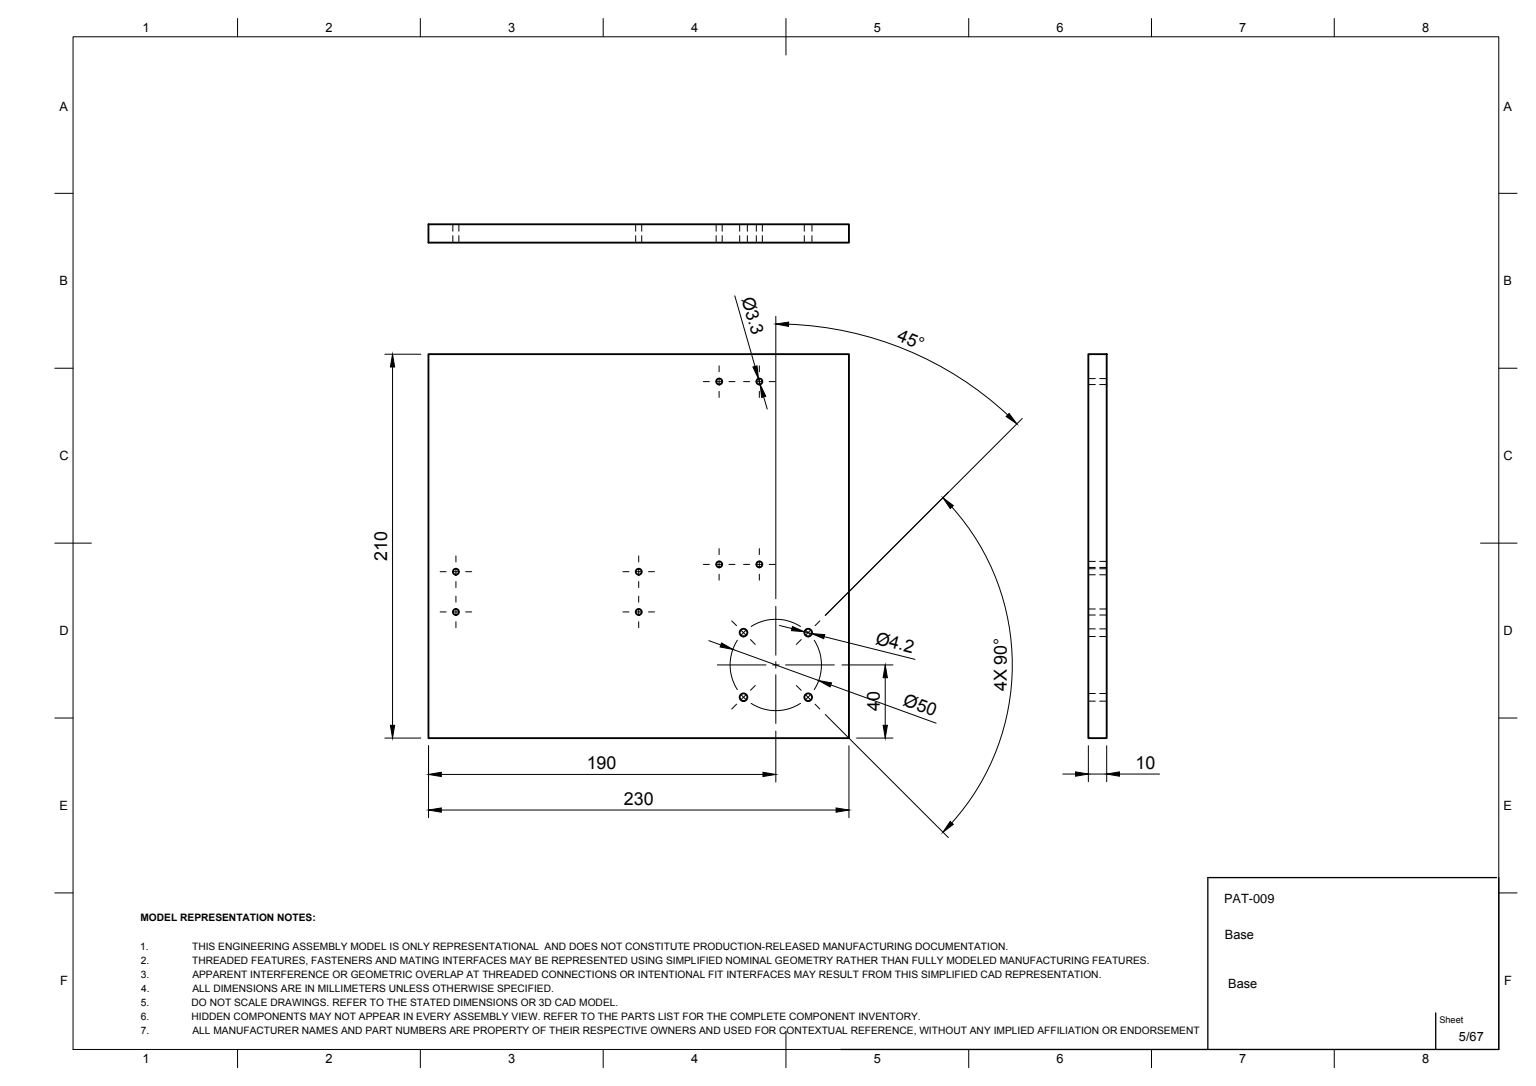
ISO-10303-21;
HEADER;
/* Generated by software containing ST-Developer
 * from STEP Tools, Inc. (www.steptools.com) 
 */

FILE_DESCRIPTION(
/* description */ ('Bell-crank linkage with push rods'),
/* implementation_level */ '2;1');

FILE_NAME(
/* name */ 'Base.step',
/* time_stamp */ '2026-10-28T03:25:15-07:00',
/* author */ (''),
/* organization */ (''),
/* preprocessor_version */ 'ST-DEVELOPER v20.2',
/* originating_system */ 'Autodesk Translation Framework v15.17.0.0',
/* authorisation */ '');

FILE_SCHEMA (('AUTOMOTIVE_DESIGN { 1 0 10303 214 3 1 1 }'));
ENDSEC;

DATA;
#10=MECHANICAL_DESIGN_GEOMETRIC_PRESENTATION_REPRESENTATION('',(#604),#16678);
#496=SHAPE_REPRESENTATION_RELATIONSHIP('SRR','None',#16912,#550);
#550=ADVANCED_BREP_SHAPE_REPRESENTATION('',(#666),#16617);
#604=STYLED_ITEM('',(#17270),#666);
#666=MANIFOLD_SOLID_BREP('Body1',#8794);
#725=FACE_BOUND('',#1786,.T.);
#726=FACE_BOUND('',#1787,.T.);
#727=FACE_BOUND('',#1788,.T.);
#728=FACE_BOUND('',#1789,.T.);
#729=FACE_BOUND('',#1790,.T.);
#730=FACE_BOUND('',#1791,.T.);
#731=FACE_BOUND('',#1792,.T.);
#732=FACE_BOUND('',#1793,.T.);
#733=FACE_BOUND('',#1794,.T.);
#734=FACE_BOUND('',#1795,.T.);
#735=FACE_BOUND('',#1796,.T.);
#736=FACE_BOUND('',#1797,.T.);
#737=FACE_BOUND('',#1799,.T.);
#738=FACE_BOUND('',#1800,.T.);
#739=FACE_BOUND('',#1801,.T.);
#740=FACE_BOUND('',#1802,.T.);
#741=FACE_BOUND('',#1803,.T.);
#742=FACE_BOUND('',#1804,.T.);
#743=FACE_BOUND('',#1805,.T.);
#744=FACE_BOUND('',#1806,.T.);
#745=FACE_BOUND('',#1807,.T.);
#746=FACE_BOUND('',#1808,.T.);
#747=FACE_BOUND('',#1809,.T.);
#748=FACE_BOUND('',#1810,.T.);
#966=PLANE('',#9493);
#967=PLANE('',#9494);
#968=PLANE('',#9495);
#969=PLANE('',#9496);
#970=PLANE('',#9497);
#971=PLANE('',#9498);
#1247=FACE_OUTER_BOUND('',#1769,.T.);
#1248=FACE_OUTER_BOUND('',#1770,.T.);
#1249=FACE_OUTER_BOUND('',#1771,.T.);
#1250=FACE_OUTER_BOUND('',#1772,.T.);
#1251=FACE_OUTER_BOUND('',#1773,.T.);
#1252=FACE_OUTER_BOUND('',#1774,.T.);
#1253=FACE_OUTER_BOUND('',#1775,.T.);
#1254=FACE_OUTER_BOUND('',#1776,.T.);
#1255=FACE_OUTER_BOUND('',#1777,.T.);
#1256=FACE_OUTER_BOUND('',#1778,.T.);
#1257=FACE_OUTER_BOUND('',#1779,.T.);
#1258=FACE_OUTER_BOUND('',#1780,.T.);
#1259=FACE_OUTER_BOUND('',#1781,.T.);
#1260=FACE_OUTER_BOUND('',#1782,.T.);
#1261=FACE_OUTER_BOUND('',#1783,.T.);
#1262=FACE_OUTER_BOUND('',#1784,.T.);
#1263=FACE_OUTER_BOUND('',#1785,.T.);
#1264=FACE_OUTER_BOUND('',#1798,.T.);
#1769=EDGE_LOOP('',(#5911,#5912,#5913,#5914));
#1770=EDGE_LOOP('',(#5915,#5916,#5917,#5918));
#1771=EDGE_LOOP('',(#5919,#5920,#5921,#5922));
#1772=EDGE_LOOP('',(#5923,#5924,#5925,#5926));
#1773=EDGE_LOOP('',(#5927,#5928,#5929,#5930));
#1774=EDGE_LOOP('',(#5931,#5932,#5933,#5934));
#1775=EDGE_LOOP('',(#5935,#5936,#5937,#5938));
#1776=EDGE_LOOP('',(#5939,#5940,#5941,#5942));
#1777=EDGE_LOOP('',(#5943,#5944,#5945,#5946));
#1778=EDGE_LOOP('',(#5947,#5948,#5949,#5950));
#1779=EDGE_LOOP('',(#5951,#5952,#5953,#5954));
#1780=EDGE_LOOP('',(#5955,#5956,#5957,#5958));
#1781=EDGE_LOOP('',(#5959,#5960,#5961,#5962));
#1782=EDGE_LOOP('',(#5963,#5964,#5965,#5966));
#1783=EDGE_LOOP('',(#5967,#5968,#5969,#5970));
#1784=EDGE_LOOP('',(#5971,#5972,#5973,#5974));
#1785=EDGE_LOOP('',(#5975,#5976,#5977,#5978));
#1786=EDGE_LOOP('',(#5979));
#1787=EDGE_LOOP('',(#5980));
#1788=EDGE_LOOP('',(#5981));
#1789=EDGE_LOOP('',(#5982));
#1790=EDGE_LOOP('',(#5983));
#1791=EDGE_LOOP('',(#5984));
#1792=EDGE_LOOP('',(#5985));
#1793=EDGE_LOOP('',(#5986));
#1794=EDGE_LOOP('',(#5987));
#1795=EDGE_LOOP('',(#5988));
#1796=EDGE_LOOP('',(#5989));
#1797=EDGE_LOOP('',(#5990));
#1798=EDGE_LOOP('',(#5991,#5992,#5993,#5994));
#1799=EDGE_LOOP('',(#5995));
#1800=EDGE_LOOP('',(#5996));
#1801=EDGE_LOOP('',(#5997));
#1802=EDGE_LOOP('',(#5998));
#1803=EDGE_LOOP('',(#5999));
#1804=EDGE_LOOP('',(#6000));
#1805=EDGE_LOOP('',(#6001));
#1806=EDGE_LOOP('',(#6002));
#1807=EDGE_LOOP('',(#6003));
#1808=EDGE_LOOP('',(#6004));
#1809=EDGE_LOOP('',(#6005));
#1810=EDGE_LOOP('',(#6006));
#2532=LINE('',#13538,#3081);
#2533=LINE('',#13544,#3082);
#2534=LINE('',#13550,#3083);
#2535=LINE('',#13556,#3084);
#2536=LINE('',#13562,#3085);
#2537=LINE('',#13568,#3086);
#2538=LINE('',#13574,#3087);
#2539=LINE('',#13580,#3088);
#2540=LINE('',#13586,#3089);
#2541=LINE('',#13592,#3090);
#2542=LINE('',#13598,#3091);
#2543=LINE('',#13604,#3092);
#2544=LINE('',#13609,#3093);
#2545=LINE('',#13611,#3094);
#2546=LINE('',#13613,#3095);
#2547=LINE('',#13614,#3096);
#2548=LINE('',#13617,#3097);
#2549=LINE('',#13619,#3098);
#2550=LINE('',#13620,#3099);
#2551=LINE('',#13623,#3100);
#2552=LINE('',#13625,#3101);
#2553=LINE('',#13626,#3102);
#2554=LINE('',#13628,#3103);
#2555=LINE('',#13629,#3104);
#3081=VECTOR('',#10640,0.165);
#3082=VECTOR('',#10647,0.165);
#3083=VECTOR('',#10654,0.165);
#3084=VECTOR('',#10661,0.165);
#3085=VECTOR('',#10668,0.164999999999999);
#3086=VECTOR('',#10675,0.164999999999999);
#3087=VECTOR('',#10682,0.165);
#3088=VECTOR('',#10689,0.165);
#3089=VECTOR('',#10696,0.21);
#3090=VECTOR('',#10703,0.21);
#3091=VECTOR('',#10710,0.21);
#3092=VECTOR('',#10717,0.21);
#3093=VECTOR('',#10722,1.);
#3094=VECTOR('',#10723,1.);
#3095=VECTOR('',#10724,1.);
#3096=VECTOR('',#10725,1.);
#3097=VECTOR('',#10728,1.);
#3098=VECTOR('',#10729,1.);
#3099=VECTOR('',#10730,1.);
#3100=VECTOR('',#10733,1.);
#3101=VECTOR('',#10734,1.);
#3102=VECTOR('',#10735,1.);
#3103=VECTOR('',#10738,1.);
#3104=VECTOR('',#10739,1.);
#3630=CIRCLE('',#9458,0.165);
#3631=CIRCLE('',#9459,0.165);
#3632=CIRCLE('',#9461,0.165);
#3633=CIRCLE('',#9462,0.165);
#3634=CIRCLE('',#9464,0.165);
#3635=CIRCLE('',#9465,0.165);
#3636=CIRCLE('',#9467,0.165);
#3637=CIRCLE('',#9468,0.165);
#3638=CIRCLE('',#9470,0.164999999999999);
#3639=CIRCLE('',#9471,0.164999999999999);
#3640=CIRCLE('',#9473,0.164999999999999);
#3641=CIRCLE('',#9474,0.164999999999999);
#3642=CIRCLE('',#9476,0.165);
#3643=CIRCLE('',#9477,0.165);
#3644=CIRCLE('',#9479,0.165);
#3645=CIRCLE('',#9480,0.165);
#3646=CIRCLE('',#9482,0.21);
#3647=CIRCLE('',#9483,0.21);
#3648=CIRCLE('',#9485,0.21);
#3649=CIRCLE('',#9486,0.21);
#3650=CIRCLE('',#9488,0.21);
#3651=CIRCLE('',#9489,0.21);
#3652=CIRCLE('',#9491,0.21);
#3653=CIRCLE('',#9492,0.21);
#4120=VERTEX_POINT('',#13535);
#4121=VERTEX_POINT('',#13537);
#4122=VERTEX_POINT('',#13541);
#4123=VERTEX_POINT('',#13543);
#4124=VERTEX_POINT('',#13547);
#4125=VERTEX_POINT('',#13549);
#4126=VERTEX_POINT('',#13553);
#4127=VERTEX_POINT('',#13555);
#4128=VERTEX_POINT('',#13559);
#4129=VERTEX_POINT('',#13561);
#4130=VERTEX_POINT('',#13565);
#4131=VERTEX_POINT('',#13567);
#4132=VERTEX_POINT('',#13571);
#4133=VERTEX_POINT('',#13573);
#4134=VERTEX_POINT('',#13577);
#4135=VERTEX_POINT('',#13579);
#4136=VERTEX_POINT('',#13583);
#4137=VERTEX_POINT('',#13585);
#4138=VERTEX_POINT('',#13589);
#4139=VERTEX_POINT('',#13591);
#4140=VERTEX_POINT('',#13595);
#4141=VERTEX_POINT('',#13597);
#4142=VERTEX_POINT('',#13601);
#4143=VERTEX_POINT('',#13603);
#4144=VERTEX_POINT('',#13607);
#4145=VERTEX_POINT('',#13608);
#4146=VERTEX_POINT('',#13610);
#4147=VERTEX_POINT('',#13612);
#4148=VERTEX_POINT('',#13616);
#4149=VERTEX_POINT('',#13618);
#4150=VERTEX_POINT('',#13622);
#4151=VERTEX_POINT('',#13624);
#4833=EDGE_CURVE('',#4120,#4120,#3630,.T.);
#4834=EDGE_CURVE('',#4120,#4121,#2532,.T.);
#4835=EDGE_CURVE('',#4121,#4121,#3631,.T.);
#4836=EDGE_CURVE('',#4122,#4122,#3632,.T.);
#4837=EDGE_CURVE('',#4122,#4123,#2533,.T.);
#4838=EDGE_CURVE('',#4123,#4123,#3633,.T.);
#4839=EDGE_CURVE('',#4124,#4124,#3634,.T.);
#4840=EDGE_CURVE('',#4124,#4125,#2534,.T.);
#4841=EDGE_CURVE('',#4125,#4125,#3635,.T.);
#4842=EDGE_CURVE('',#4126,#4126,#3636,.T.);
#4843=EDGE_CURVE('',#4126,#4127,#2535,.T.);
#4844=EDGE_CURVE('',#4127,#4127,#3637,.T.);
#4845=EDGE_CURVE('',#4128,#4128,#3638,.T.);
#4846=EDGE_CURVE('',#4128,#4129,#2536,.T.);
#4847=EDGE_CURVE('',#4129,#4129,#3639,.T.);
#4848=EDGE_CURVE('',#4130,#4130,#3640,.T.);
#4849=EDGE_CURVE('',#4130,#4131,#2537,.T.);
#4850=EDGE_CURVE('',#4131,#4131,#3641,.T.);
#4851=EDGE_CURVE('',#4132,#4132,#3642,.T.);
#4852=EDGE_CURVE('',#4132,#4133,#2538,.T.);
#4853=EDGE_CURVE('',#4133,#4133,#3643,.T.);
#4854=EDGE_CURVE('',#4134,#4134,#3644,.T.);
#4855=EDGE_CURVE('',#4134,#4135,#2539,.T.);
#4856=EDGE_CURVE('',#4135,#4135,#3645,.T.);
#4857=EDGE_CURVE('',#4136,#4136,#3646,.T.);
#4858=EDGE_CURVE('',#4136,#4137,#2540,.T.);
#4859=EDGE_CURVE('',#4137,#4137,#3647,.T.);
#4860=EDGE_CURVE('',#4138,#4138,#3648,.T.);
#4861=EDGE_CURVE('',#4138,#4139,#2541,.T.);
#4862=EDGE_CURVE('',#4139,#4139,#3649,.T.);
#4863=EDGE_CURVE('',#4140,#4140,#3650,.T.);
#4864=EDGE_CURVE('',#4140,#4141,#2542,.T.);
#4865=EDGE_CURVE('',#4141,#4141,#3651,.T.);
#4866=EDGE_CURVE('',#4142,#4142,#3652,.T.);
#4867=EDGE_CURVE('',#4142,#4143,#2543,.T.);
#4868=EDGE_CURVE('',#4143,#4143,#3653,.T.);
#4869=EDGE_CURVE('',#4144,#4145,#2544,.T.);
#4870=EDGE_CURVE('',#4145,#4146,#2545,.T.);
#4871=EDGE_CURVE('',#4147,#4146,#2546,.T.);
#4872=EDGE_CURVE('',#4144,#4147,#2547,.T.);
#4873=EDGE_CURVE('',#4148,#4144,#2548,.T.);
#4874=EDGE_CURVE('',#4149,#4147,#2549,.T.);
#4875=EDGE_CURVE('',#4148,#4149,#2550,.T.);
#4876=EDGE_CURVE('',#4150,#4148,#2551,.T.);
#4877=EDGE_CURVE('',#4151,#4149,#2552,.T.);
#4878=EDGE_CURVE('',#4150,#4151,#2553,.T.);
#4879=EDGE_CURVE('',#4145,#4150,#2554,.T.);
#4880=EDGE_CURVE('',#4146,#4151,#2555,.T.);
#5911=ORIENTED_EDGE('',*,*,#4833,.F.);
#5912=ORIENTED_EDGE('',*,*,#4834,.T.);
#5913=ORIENTED_EDGE('',*,*,#4835,.F.);
#5914=ORIENTED_EDGE('',*,*,#4834,.F.);
#5915=ORIENTED_EDGE('',*,*,#4836,.F.);
#5916=ORIENTED_EDGE('',*,*,#4837,.T.);
#5917=ORIENTED_EDGE('',*,*,#4838,.F.);
#5918=ORIENTED_EDGE('',*,*,#4837,.F.);
#5919=ORIENTED_EDGE('',*,*,#4839,.F.);
#5920=ORIENTED_EDGE('',*,*,#4840,.T.);
#5921=ORIENTED_EDGE('',*,*,#4841,.F.);
#5922=ORIENTED_EDGE('',*,*,#4840,.F.);
#5923=ORIENTED_EDGE('',*,*,#4842,.F.);
#5924=ORIENTED_EDGE('',*,*,#4843,.T.);
#5925=ORIENTED_EDGE('',*,*,#4844,.F.);
#5926=ORIENTED_EDGE('',*,*,#4843,.F.);
#5927=ORIENTED_EDGE('',*,*,#4845,.F.);
#5928=ORIENTED_EDGE('',*,*,#4846,.T.);
#5929=ORIENTED_EDGE('',*,*,#4847,.F.);
#5930=ORIENTED_EDGE('',*,*,#4846,.F.);
#5931=ORIENTED_EDGE('',*,*,#4848,.F.);
#5932=ORIENTED_EDGE('',*,*,#4849,.T.);
#5933=ORIENTED_EDGE('',*,*,#4850,.F.);
#5934=ORIENTED_EDGE('',*,*,#4849,.F.);
#5935=ORIENTED_EDGE('',*,*,#4851,.F.);
#5936=ORIENTED_EDGE('',*,*,#4852,.T.);
#5937=ORIENTED_EDGE('',*,*,#4853,.F.);
#5938=ORIENTED_EDGE('',*,*,#4852,.F.);
#5939=ORIENTED_EDGE('',*,*,#4854,.F.);
#5940=ORIENTED_EDGE('',*,*,#4855,.T.);
#5941=ORIENTED_EDGE('',*,*,#4856,.F.);
#5942=ORIENTED_EDGE('',*,*,#4855,.F.);
#5943=ORIENTED_EDGE('',*,*,#4857,.F.);
#5944=ORIENTED_EDGE('',*,*,#4858,.T.);
#5945=ORIENTED_EDGE('',*,*,#4859,.F.);
#5946=ORIENTED_EDGE('',*,*,#4858,.F.);
#5947=ORIENTED_EDGE('',*,*,#4860,.F.);
#5948=ORIENTED_EDGE('',*,*,#4861,.T.);
#5949=ORIENTED_EDGE('',*,*,#4862,.F.);
#5950=ORIENTED_EDGE('',*,*,#4861,.F.);
#5951=ORIENTED_EDGE('',*,*,#4863,.F.);
#5952=ORIENTED_EDGE('',*,*,#4864,.T.);
#5953=ORIENTED_EDGE('',*,*,#4865,.F.);
#5954=ORIENTED_EDGE('',*,*,#4864,.F.);
#5955=ORIENTED_EDGE('',*,*,#4866,.F.);
#5956=ORIENTED_EDGE('',*,*,#4867,.T.);
#5957=ORIENTED_EDGE('',*,*,#4868,.F.);
#5958=ORIENTED_EDGE('',*,*,#4867,.F.);
#5959=ORIENTED_EDGE('',*,*,#4869,.T.);
#5960=ORIENTED_EDGE('',*,*,#4870,.T.);
#5961=ORIENTED_EDGE('',*,*,#4871,.F.);
#5962=ORIENTED_EDGE('',*,*,#4872,.F.);
#5963=ORIENTED_EDGE('',*,*,#4873,.T.);
#5964=ORIENTED_EDGE('',*,*,#4872,.T.);
#5965=ORIENTED_EDGE('',*,*,#4874,.F.);
#5966=ORIENTED_EDGE('',*,*,#4875,.F.);
#5967=ORIENTED_EDGE('',*,*,#4876,.T.);
#5968=ORIENTED_EDGE('',*,*,#4875,.T.);
#5969=ORIENTED_EDGE('',*,*,#4877,.F.);
#5970=ORIENTED_EDGE('',*,*,#4878,.F.);
#5971=ORIENTED_EDGE('',*,*,#4879,.T.);
#5972=ORIENTED_EDGE('',*,*,#4878,.T.);
#5973=ORIENTED_EDGE('',*,*,#4880,.F.);
#5974=ORIENTED_EDGE('',*,*,#4870,.F.);
#5975=ORIENTED_EDGE('',*,*,#4880,.T.);
#5976=ORIENTED_EDGE('',*,*,#4877,.T.);
#5977=ORIENTED_EDGE('',*,*,#4874,.T.);
#5978=ORIENTED_EDGE('',*,*,#4871,.T.);
#5979=ORIENTED_EDGE('',*,*,#4841,.T.);
#5980=ORIENTED_EDGE('',*,*,#4844,.T.);
#5981=ORIENTED_EDGE('',*,*,#4868,.T.);
#5982=ORIENTED_EDGE('',*,*,#4865,.T.);
#5983=ORIENTED_EDGE('',*,*,#4862,.T.);
#5984=ORIENTED_EDGE('',*,*,#4859,.T.);
#5985=ORIENTED_EDGE('',*,*,#4856,.T.);
#5986=ORIENTED_EDGE('',*,*,#4853,.T.);
#5987=ORIENTED_EDGE('',*,*,#4850,.T.);
#5988=ORIENTED_EDGE('',*,*,#4847,.T.);
#5989=ORIENTED_EDGE('',*,*,#4838,.T.);
#5990=ORIENTED_EDGE('',*,*,#4835,.T.);
#5991=ORIENTED_EDGE('',*,*,#4879,.F.);
#5992=ORIENTED_EDGE('',*,*,#4869,.F.);
#5993=ORIENTED_EDGE('',*,*,#4873,.F.);
#5994=ORIENTED_EDGE('',*,*,#4876,.F.);
#5995=ORIENTED_EDGE('',*,*,#4839,.T.);
#5996=ORIENTED_EDGE('',*,*,#4842,.T.);
#5997=ORIENTED_EDGE('',*,*,#4866,.T.);
#5998=ORIENTED_EDGE('',*,*,#4863,.T.);
#5999=ORIENTED_EDGE('',*,*,#4860,.T.);
#6000=ORIENTED_EDGE('',*,*,#4857,.T.);
#6001=ORIENTED_EDGE('',*,*,#4854,.T.);
#6002=ORIENTED_EDGE('',*,*,#4851,.T.);
#6003=ORIENTED_EDGE('',*,*,#4848,.T.);
#6004=ORIENTED_EDGE('',*,*,#4845,.T.);
#6005=ORIENTED_EDGE('',*,*,#4836,.T.);
#6006=ORIENTED_EDGE('',*,*,#4833,.T.);
#8067=CYLINDRICAL_SURFACE('',#9457,0.165);
#8068=CYLINDRICAL_SURFACE('',#9460,0.165);
#8069=CYLINDRICAL_SURFACE('',#9463,0.165);
#8070=CYLINDRICAL_SURFACE('',#9466,0.165);
#8071=CYLINDRICAL_SURFACE('',#9469,0.164999999999999);
#8072=CYLINDRICAL_SURFACE('',#9472,0.164999999999999);
#8073=CYLINDRICAL_SURFACE('',#9475,0.165);
#8074=CYLINDRICAL_SURFACE('',#9478,0.165);
#8075=CYLINDRICAL_SURFACE('',#9481,0.21);
#8076=CYLINDRICAL_SURFACE('',#9484,0.21);
#8077=CYLINDRICAL_SURFACE('',#9487,0.21);
#8078=CYLINDRICAL_SURFACE('',#9490,0.21);
#8272=ADVANCED_FACE('',(#1247),#8067,.F.);
#8273=ADVANCED_FACE('',(#1248),#8068,.F.);
#8274=ADVANCED_FACE('',(#1249),#8069,.F.);
#8275=ADVANCED_FACE('',(#1250),#8070,.F.);
#8276=ADVANCED_FACE('',(#1251),#8071,.F.);
#8277=ADVANCED_FACE('',(#1252),#8072,.F.);
#8278=ADVANCED_FACE('',(#1253),#8073,.F.);
#8279=ADVANCED_FACE('',(#1254),#8074,.F.);
#8280=ADVANCED_FACE('',(#1255),#8075,.F.);
#8281=ADVANCED_FACE('',(#1256),#8076,.F.);
#8282=ADVANCED_FACE('',(#1257),#8077,.F.);
#8283=ADVANCED_FACE('',(#1258),#8078,.F.);
#8284=ADVANCED_FACE('',(#1259),#966,.T.);
#8285=ADVANCED_FACE('',(#1260),#967,.T.);
#8286=ADVANCED_FACE('',(#1261),#968,.T.);
#8287=ADVANCED_FACE('',(#1262),#969,.T.);
#8288=ADVANCED_FACE('',(#1263,#725,#726,#727,#728,#729,#730,#731,#732,#733,
#734,#735,#736),#970,.T.);
#8289=ADVANCED_FACE('',(#1264,#737,#738,#739,#740,#741,#742,#743,#744,#745,
#746,#747,#748),#971,.F.);
#8794=CLOSED_SHELL('',(#8272,#8273,#8274,#8275,#8276,#8277,#8278,#8279,
#8280,#8281,#8282,#8283,#8284,#8285,#8286,#8287,#8288,#8289));
#9456=AXIS2_PLACEMENT_3D('',#13533,#10634,#10635);
#9457=AXIS2_PLACEMENT_3D('',#13534,#10636,#10637);
#9458=AXIS2_PLACEMENT_3D('',#13536,#10638,#10639);
#9459=AXIS2_PLACEMENT_3D('',#13539,#10641,#10642);
#9460=AXIS2_PLACEMENT_3D('',#13540,#10643,#10644);
#9461=AXIS2_PLACEMENT_3D('',#13542,#10645,#10646);
#9462=AXIS2_PLACEMENT_3D('',#13545,#10648,#10649);
#9463=AXIS2_PLACEMENT_3D('',#13546,#10650,#10651);
#9464=AXIS2_PLACEMENT_3D('',#13548,#10652,#10653);
#9465=AXIS2_PLACEMENT_3D('',#13551,#10655,#10656);
#9466=AXIS2_PLACEMENT_3D('',#13552,#10657,#10658);
#9467=AXIS2_PLACEMENT_3D('',#13554,#10659,#10660);
#9468=AXIS2_PLACEMENT_3D('',#13557,#10662,#10663);
#9469=AXIS2_PLACEMENT_3D('',#13558,#10664,#10665);
#9470=AXIS2_PLACEMENT_3D('',#13560,#10666,#10667);
#9471=AXIS2_PLACEMENT_3D('',#13563,#10669,#10670);
#9472=AXIS2_PLACEMENT_3D('',#13564,#10671,#10672);
#9473=AXIS2_PLACEMENT_3D('',#13566,#10673,#10674);
#9474=AXIS2_PLACEMENT_3D('',#13569,#10676,#10677);
#9475=AXIS2_PLACEMENT_3D('',#13570,#10678,#10679);
#9476=AXIS2_PLACEMENT_3D('',#13572,#10680,#10681);
#9477=AXIS2_PLACEMENT_3D('',#13575,#10683,#10684);
#9478=AXIS2_PLACEMENT_3D('',#13576,#10685,#10686);
#9479=AXIS2_PLACEMENT_3D('',#13578,#10687,#10688);
#9480=AXIS2_PLACEMENT_3D('',#13581,#10690,#10691);
#9481=AXIS2_PLACEMENT_3D('',#13582,#10692,#10693);
#9482=AXIS2_PLACEMENT_3D('',#13584,#10694,#10695);
#9483=AXIS2_PLACEMENT_3D('',#13587,#10697,#10698);
#9484=AXIS2_PLACEMENT_3D('',#13588,#10699,#10700);
#9485=AXIS2_PLACEMENT_3D('',#13590,#10701,#10702);
#9486=AXIS2_PLACEMENT_3D('',#13593,#10704,#10705);
#9487=AXIS2_PLACEMENT_3D('',#13594,#10706,#10707);
#9488=AXIS2_PLACEMENT_3D('',#13596,#10708,#10709);
#9489=AXIS2_PLACEMENT_3D('',#13599,#10711,#10712);
#9490=AXIS2_PLACEMENT_3D('',#13600,#10713,#10714);
#9491=AXIS2_PLACEMENT_3D('',#13602,#10715,#10716);
#9492=AXIS2_PLACEMENT_3D('',#13605,#10718,#10719);
#9493=AXIS2_PLACEMENT_3D('',#13606,#10720,#10721);
#9494=AXIS2_PLACEMENT_3D('',#13615,#10726,#10727);
#9495=AXIS2_PLACEMENT_3D('',#13621,#10731,#10732);
#9496=AXIS2_PLACEMENT_3D('',#13627,#10736,#10737);
#9497=AXIS2_PLACEMENT_3D('',#13630,#10740,#10741);
#9498=AXIS2_PLACEMENT_3D('',#13631,#10742,#10743);
#10634=DIRECTION('axis',(0.,0.,1.));
#10635=DIRECTION('refdir',(1.,0.,0.));
#10636=DIRECTION('center_axis',(0.,0.,1.));
#10637=DIRECTION('ref_axis',(1.,0.,0.));
#10638=DIRECTION('center_axis',(0.,0.,1.));
#10639=DIRECTION('ref_axis',(1.,0.,0.));
#10640=DIRECTION('',(0.,0.,1.));
#10641=DIRECTION('center_axis',(0.,0.,-1.));
#10642=DIRECTION('ref_axis',(1.,0.,0.));
#10643=DIRECTION('center_axis',(0.,0.,1.));
#10644=DIRECTION('ref_axis',(1.,0.,0.));
#10645=DIRECTION('center_axis',(0.,0.,1.));
#10646=DIRECTION('ref_axis',(1.,0.,0.));
#10647=DIRECTION('',(0.,0.,1.));
#10648=DIRECTION('center_axis',(0.,0.,-1.));
#10649=DIRECTION('ref_axis',(1.,0.,0.));
#10650=DIRECTION('center_axis',(0.,0.,1.));
#10651=DIRECTION('ref_axis',(1.,0.,0.));
#10652=DIRECTION('center_axis',(0.,0.,1.));
#10653=DIRECTION('ref_axis',(1.,0.,0.));
#10654=DIRECTION('',(0.,0.,1.));
#10655=DIRECTION('center_axis',(0.,0.,-1.));
#10656=DIRECTION('ref_axis',(1.,0.,0.));
#10657=DIRECTION('center_axis',(0.,0.,1.));
#10658=DIRECTION('ref_axis',(1.,0.,0.));
#10659=DIRECTION('center_axis',(0.,0.,1.));
#10660=DIRECTION('ref_axis',(1.,0.,0.));
#10661=DIRECTION('',(0.,0.,1.));
#10662=DIRECTION('center_axis',(0.,0.,-1.));
#10663=DIRECTION('ref_axis',(1.,0.,0.));
#10664=DIRECTION('center_axis',(0.,0.,1.));
#10665=DIRECTION('ref_axis',(1.,0.,0.));
#10666=DIRECTION('center_axis',(0.,0.,1.));
#10667=DIRECTION('ref_axis',(1.,0.,0.));
#10668=DIRECTION('',(0.,0.,1.));
#10669=DIRECTION('center_axis',(0.,0.,-1.));
#10670=DIRECTION('ref_axis',(1.,0.,0.));
#10671=DIRECTION('center_axis',(0.,0.,1.));
#10672=DIRECTION('ref_axis',(1.,0.,0.));
#10673=DIRECTION('center_axis',(0.,0.,1.));
#10674=DIRECTION('ref_axis',(1.,0.,0.));
#10675=DIRECTION('',(0.,0.,1.));
#10676=DIRECTION('center_axis',(0.,0.,-1.));
#10677=DIRECTION('ref_axis',(1.,0.,0.));
#10678=DIRECTION('center_axis',(0.,0.,1.));
#10679=DIRECTION('ref_axis',(1.,0.,0.));
#10680=DIRECTION('center_axis',(0.,0.,1.));
#10681=DIRECTION('ref_axis',(1.,0.,0.));
#10682=DIRECTION('',(0.,0.,1.));
#10683=DIRECTION('center_axis',(0.,0.,-1.));
#10684=DIRECTION('ref_axis',(1.,0.,0.));
#10685=DIRECTION('center_axis',(0.,0.,1.));
#10686=DIRECTION('ref_axis',(1.,0.,0.));
#10687=DIRECTION('center_axis',(0.,0.,1.));
#10688=DIRECTION('ref_axis',(1.,0.,0.));
#10689=DIRECTION('',(0.,0.,1.));
#10690=DIRECTION('center_axis',(0.,0.,-1.));
#10691=DIRECTION('ref_axis',(1.,0.,0.));
#10692=DIRECTION('center_axis',(0.,0.,1.));
#10693=DIRECTION('ref_axis',(1.,0.,0.));
#10694=DIRECTION('center_axis',(0.,0.,1.));
#10695=DIRECTION('ref_axis',(1.,0.,0.));
#10696=DIRECTION('',(0.,0.,1.));
#10697=DIRECTION('center_axis',(0.,0.,-1.));
#10698=DIRECTION('ref_axis',(1.,0.,0.));
#10699=DIRECTION('center_axis',(0.,0.,1.));
#10700=DIRECTION('ref_axis',(1.,0.,0.));
#10701=DIRECTION('center_axis',(0.,0.,1.));
#10702=DIRECTION('ref_axis',(1.,0.,0.));
#10703=DIRECTION('',(0.,0.,1.));
#10704=DIRECTION('center_axis',(0.,0.,-1.));
#10705=DIRECTION('ref_axis',(1.,0.,0.));
#10706=DIRECTION('center_axis',(0.,0.,1.));
#10707=DIRECTION('ref_axis',(1.,0.,0.));
#10708=DIRECTION('center_axis',(0.,0.,1.));
#10709=DIRECTION('ref_axis',(1.,0.,0.));
#10710=DIRECTION('',(0.,0.,1.));
#10711=DIRECTION('center_axis',(0.,0.,-1.));
#10712=DIRECTION('ref_axis',(1.,0.,0.));
#10713=DIRECTION('center_axis',(0.,0.,1.));
#10714=DIRECTION('ref_axis',(1.,0.,0.));
#10715=DIRECTION('center_axis',(0.,0.,1.));
#10716=DIRECTION('ref_axis',(1.,0.,0.));
#10717=DIRECTION('',(0.,0.,1.));
#10718=DIRECTION('center_axis',(0.,0.,-1.));
#10719=DIRECTION('ref_axis',(1.,0.,0.));
#10720=DIRECTION('center_axis',(0.,1.,0.));
#10721=DIRECTION('ref_axis',(-1.,0.,0.));
#10722=DIRECTION('',(-1.,0.,0.));
#10723=DIRECTION('',(0.,0.,1.));
#10724=DIRECTION('',(-1.,0.,0.));
#10725=DIRECTION('',(0.,0.,1.));
#10726=DIRECTION('center_axis',(1.,0.,0.));
#10727=DIRECTION('ref_axis',(0.,1.,0.));
#10728=DIRECTION('',(0.,1.,0.));
#10729=DIRECTION('',(0.,1.,0.));
#10730=DIRECTION('',(0.,0.,1.));
#10731=DIRECTION('center_axis',(0.,-1.,0.));
#10732=DIRECTION('ref_axis',(1.,0.,0.));
#10733=DIRECTION('',(1.,0.,0.));
#10734=DIRECTION('',(1.,0.,0.));
#10735=DIRECTION('',(0.,0.,1.));
#10736=DIRECTION('center_axis',(-1.,0.,0.));
#10737=DIRECTION('ref_axis',(0.,-1.,0.));
#10738=DIRECTION('',(0.,-1.,0.));
#10739=DIRECTION('',(0.,-1.,0.));
#10740=DIRECTION('center_axis',(0.,0.,1.));
#10741=DIRECTION('ref_axis',(1.,0.,0.));
#10742=DIRECTION('center_axis',(0.,0.,1.));
#10743=DIRECTION('ref_axis',(1.,0.,0.));
#13533=CARTESIAN_POINT('',(0.,0.,0.));
#13534=CARTESIAN_POINT('Origin',(2.9,17.5,-0.1));
#13535=CARTESIAN_POINT('',(2.735,17.5,0.));
#13536=CARTESIAN_POINT('Origin',(2.9,17.5,0.));
#13537=CARTESIAN_POINT('',(2.735,17.5,1.));
#13538=CARTESIAN_POINT('',(2.735,17.5,-0.1));
#13539=CARTESIAN_POINT('Origin',(2.9,17.5,1.));
#13540=CARTESIAN_POINT('Origin',(5.1,17.5,-0.1));
#13541=CARTESIAN_POINT('',(4.935,17.5,0.));
#13542=CARTESIAN_POINT('Origin',(5.1,17.5,0.));
#13543=CARTESIAN_POINT('',(4.935,17.5,1.));
#13544=CARTESIAN_POINT('',(4.935,17.5,-0.1));
#13545=CARTESIAN_POINT('Origin',(5.1,17.5,1.));
#13546=CARTESIAN_POINT('Origin',(2.9,7.5,-0.1));
#13547=CARTESIAN_POINT('',(2.735,7.5,0.));
#13548=CARTESIAN_POINT('Origin',(2.9,7.5,0.));
#13549=CARTESIAN_POINT('',(2.735,7.5,1.));
#13550=CARTESIAN_POINT('',(2.735,7.5,-0.1));
#13551=CARTESIAN_POINT('Origin',(2.9,7.5,1.));
#13552=CARTESIAN_POINT('Origin',(5.1,7.5,-0.1));
#13553=CARTESIAN_POINT('',(4.935,7.5,0.));
#13554=CARTESIAN_POINT('Origin',(5.1,7.5,0.));
#13555=CARTESIAN_POINT('',(4.935,7.5,1.));
#13556=CARTESIAN_POINT('',(4.935,7.5,-0.1));
#13557=CARTESIAN_POINT('Origin',(5.1,7.5,1.));
#13558=CARTESIAN_POINT('Origin',(15.5,0.9,-0.1));
#13559=CARTESIAN_POINT('',(15.335,0.9,0.));
#13560=CARTESIAN_POINT('Origin',(15.5,0.9,0.));
#13561=CARTESIAN_POINT('',(15.335,0.9,1.));
#13562=CARTESIAN_POINT('',(15.335,0.9,-0.1));
#13563=CARTESIAN_POINT('Origin',(15.5,0.9,1.));
#13564=CARTESIAN_POINT('Origin',(15.5,3.1,-0.1));
#13565=CARTESIAN_POINT('',(15.335,3.1,0.));
#13566=CARTESIAN_POINT('Origin',(15.5,3.1,0.));
#13567=CARTESIAN_POINT('',(15.335,3.1,1.));
#13568=CARTESIAN_POINT('',(15.335,3.1,-0.1));
#13569=CARTESIAN_POINT('Origin',(15.5,3.1,1.));
#13570=CARTESIAN_POINT('Origin',(5.5,0.9,-0.1));
#13571=CARTESIAN_POINT('',(5.335,0.9,0.));
#13572=CARTESIAN_POINT('Origin',(5.5,0.9,0.));
#13573=CARTESIAN_POINT('',(5.335,0.9,1.));
#13574=CARTESIAN_POINT('',(5.335,0.9,-0.1));
#13575=CARTESIAN_POINT('Origin',(5.5,0.9,1.));
#13576=CARTESIAN_POINT('Origin',(5.5,3.1,-0.1));
#13577=CARTESIAN_POINT('',(5.335,3.1,0.));
#13578=CARTESIAN_POINT('Origin',(5.5,3.1,0.));
#13579=CARTESIAN_POINT('',(5.335,3.1,1.));
#13580=CARTESIAN_POINT('',(5.335,3.1,-0.1));
#13581=CARTESIAN_POINT('Origin',(5.5,3.1,1.));
#13582=CARTESIAN_POINT('Origin',(-1.76776695296637,-1.76776695296637,-0.1));
#13583=CARTESIAN_POINT('',(-1.97776695296637,-1.76776695296637,0.));
#13584=CARTESIAN_POINT('Origin',(-1.76776695296637,-1.76776695296637,0.));
#13585=CARTESIAN_POINT('',(-1.97776695296637,-1.76776695296637,1.));
#13586=CARTESIAN_POINT('',(-1.97776695296637,-1.76776695296637,-0.1));
#13587=CARTESIAN_POINT('Origin',(-1.76776695296637,-1.76776695296637,1.));
#13588=CARTESIAN_POINT('Origin',(-1.76776695296637,1.76776695296637,-0.1));
#13589=CARTESIAN_POINT('',(-1.97776695296637,1.76776695296637,0.));
#13590=CARTESIAN_POINT('Origin',(-1.76776695296637,1.76776695296637,0.));
#13591=CARTESIAN_POINT('',(-1.97776695296637,1.76776695296637,1.));
#13592=CARTESIAN_POINT('',(-1.97776695296637,1.76776695296637,-0.1));
#13593=CARTESIAN_POINT('Origin',(-1.76776695296637,1.76776695296637,1.));
#13594=CARTESIAN_POINT('Origin',(1.76776695296637,1.76776695296637,-0.1));
#13595=CARTESIAN_POINT('',(1.55776695296637,1.76776695296637,0.));
#13596=CARTESIAN_POINT('Origin',(1.76776695296637,1.76776695296637,0.));
#13597=CARTESIAN_POINT('',(1.55776695296637,1.76776695296637,1.));
#13598=CARTESIAN_POINT('',(1.55776695296637,1.76776695296637,-0.1));
#13599=CARTESIAN_POINT('Origin',(1.76776695296637,1.76776695296637,1.));
#13600=CARTESIAN_POINT('Origin',(1.76776695296637,-1.76776695296637,-0.1));
#13601=CARTESIAN_POINT('',(1.55776695296637,-1.76776695296637,0.));
#13602=CARTESIAN_POINT('Origin',(1.76776695296637,-1.76776695296637,0.));
#13603=CARTESIAN_POINT('',(1.55776695296637,-1.76776695296637,1.));
#13604=CARTESIAN_POINT('',(1.55776695296637,-1.76776695296637,-0.1));
#13605=CARTESIAN_POINT('Origin',(1.76776695296637,-1.76776695296637,1.));
#13606=CARTESIAN_POINT('Origin',(17.,19.,0.));
#13607=CARTESIAN_POINT('',(17.,19.,0.));
#13608=CARTESIAN_POINT('',(-4.,19.,0.));
#13609=CARTESIAN_POINT('',(17.,19.,0.));
#13610=CARTESIAN_POINT('',(-4.,19.,1.));
#13611=CARTESIAN_POINT('',(-4.,19.,0.));
#13612=CARTESIAN_POINT('',(17.,19.,1.));
#13613=CARTESIAN_POINT('',(17.,19.,1.));
#13614=CARTESIAN_POINT('',(17.,19.,0.));
#13615=CARTESIAN_POINT('Origin',(17.,-4.,0.));
#13616=CARTESIAN_POINT('',(17.,-4.,0.));
#13617=CARTESIAN_POINT('',(17.,-4.,0.));
#13618=CARTESIAN_POINT('',(17.,-4.,1.));
#13619=CARTESIAN_POINT('',(17.,-4.,1.));
#13620=CARTESIAN_POINT('',(17.,-4.,0.));
#13621=CARTESIAN_POINT('Origin',(-4.,-4.,0.));
#13622=CARTESIAN_POINT('',(-4.,-4.,0.));
#13623=CARTESIAN_POINT('',(-4.,-4.,0.));
#13624=CARTESIAN_POINT('',(-4.,-4.,1.));
#13625=CARTESIAN_POINT('',(-4.,-4.,1.));
#13626=CARTESIAN_POINT('',(-4.,-4.,0.));
#13627=CARTESIAN_POINT('Origin',(-4.,19.,0.));
#13628=CARTESIAN_POINT('',(-4.,19.,0.));
#13629=CARTESIAN_POINT('',(-4.,19.,1.));
#13630=CARTESIAN_POINT('Origin',(6.5,7.5,1.));
#13631=CARTESIAN_POINT('Origin',(6.5,7.5,0.));
#16553=UNCERTAINTY_MEASURE_WITH_UNIT(LENGTH_MEASURE(0.001),#16679,
'DISTANCE_ACCURACY_VALUE',
'Maximum model space distance between geometric entities at asserted c
onnectivities');
#16614=UNCERTAINTY_MEASURE_WITH_UNIT(LENGTH_MEASURE(0.001),#16679,
'DISTANCE_ACCURACY_VALUE',
'Maximum model space distance between geometric entities at asserted c
onnectivities');
#16617=(
GEOMETRIC_REPRESENTATION_CONTEXT(3)
GLOBAL_UNCERTAINTY_ASSIGNED_CONTEXT((#16553))
GLOBAL_UNIT_ASSIGNED_CONTEXT((#16679,#16681,#16682))
REPRESENTATION_CONTEXT('','3D')
);
#16678=(
GEOMETRIC_REPRESENTATION_CONTEXT(3)
GLOBAL_UNCERTAINTY_ASSIGNED_CONTEXT((#16614))
GLOBAL_UNIT_ASSIGNED_CONTEXT((#16679,#16681,#16682))
REPRESENTATION_CONTEXT('','3D')
);
#16679=(
LENGTH_UNIT()
NAMED_UNIT(*)
SI_UNIT(.CENTI.,.METRE.)
);
#16681=(
NAMED_UNIT(*)
PLANE_ANGLE_UNIT()
SI_UNIT($,.RADIAN.)
);
#16682=(
NAMED_UNIT(*)
SI_UNIT($,.STERADIAN.)
SOLID_ANGLE_UNIT()
);
#16685=SHAPE_DEFINITION_REPRESENTATION(#16748,#16912);
#16748=PRODUCT_DEFINITION_SHAPE('',$,#16976);
#16912=SHAPE_REPRESENTATION('',(#9456),#16617);
#16973=PRODUCT_DEFINITION_CONTEXT('part definition',#17164,'design');
#16976=PRODUCT_DEFINITION('Base','Base',#17039,#16973);
#17039=PRODUCT_DEFINITION_FORMATION('',$,#17168);
#17164=APPLICATION_CONTEXT(
'Core Data for Automotive Mechanical Design Process');
#17165=PRODUCT_CONTEXT('part definition',#17164,'mechanical');
#17168=PRODUCT('Base','Base','Base',(#17165));
#17264=COLOUR_RGB('Dark Blue',0.08,0.2,0.34);
#17265=FILL_AREA_STYLE_COLOUR('',#17264);
#17266=FILL_AREA_STYLE('',(#17265));
#17267=SURFACE_STYLE_FILL_AREA(#17266);
#17268=SURFACE_SIDE_STYLE('',(#17267));
#17269=SURFACE_STYLE_USAGE(.BOTH.,#17268);
#17270=PRESENTATION_STYLE_ASSIGNMENT((#17269));
ENDSEC;
END-ISO-10303-21;
